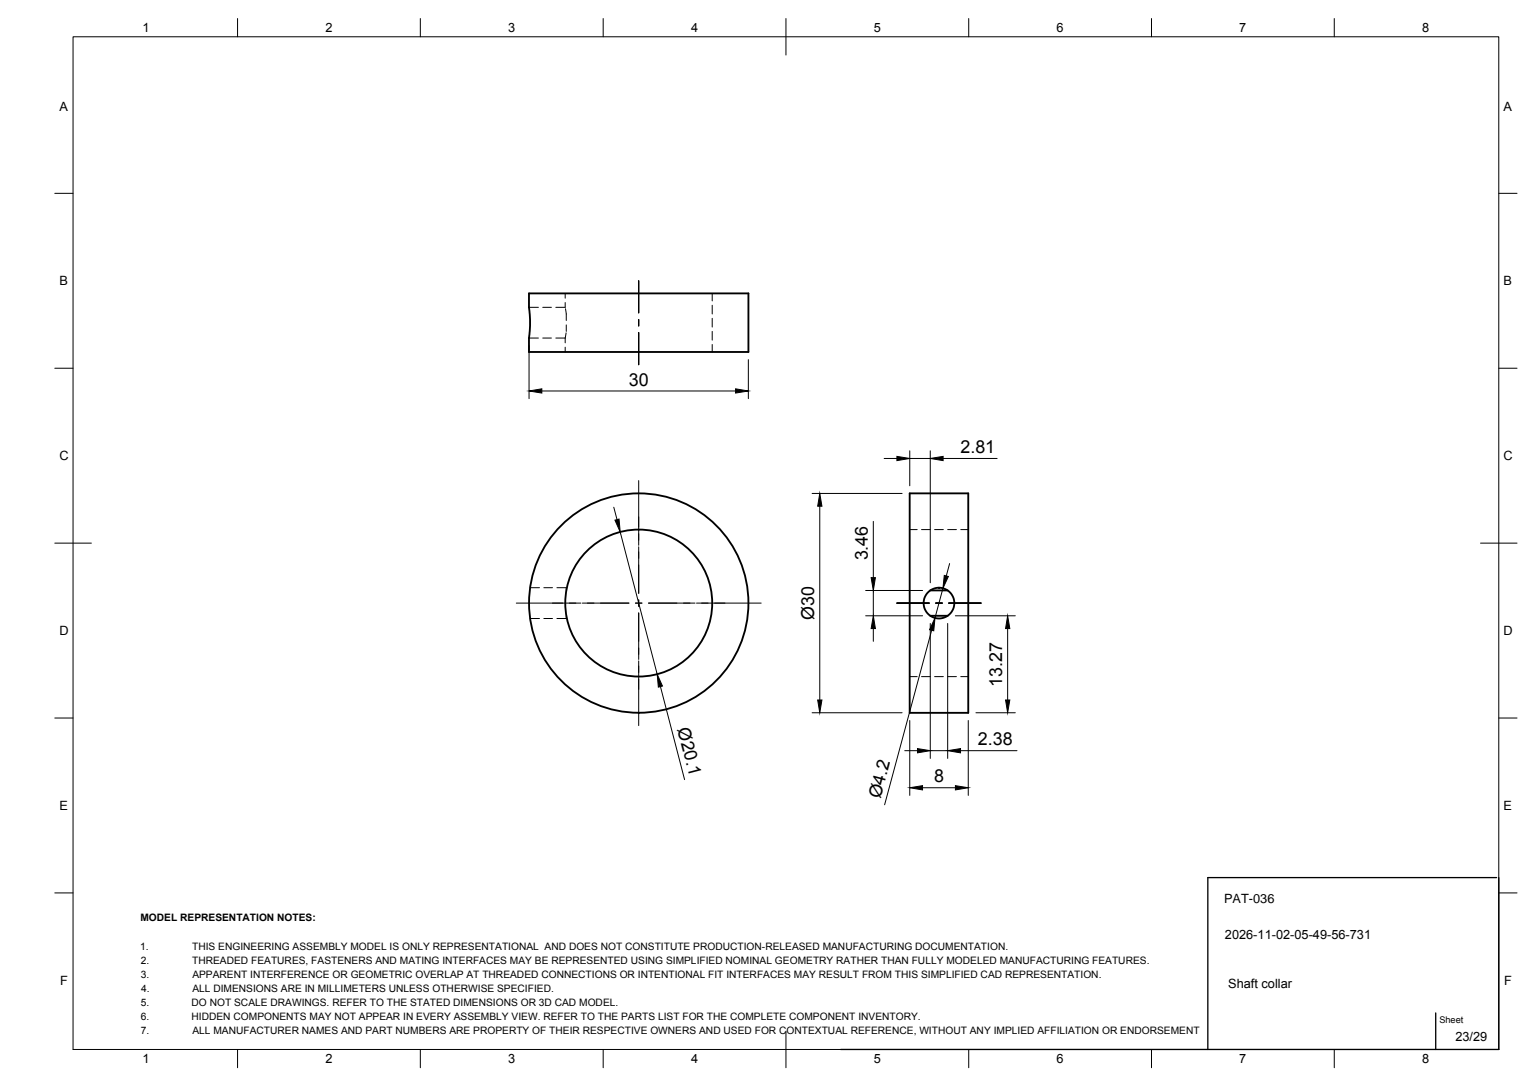
ISO-10303-21;
HEADER;
/* Generated by software containing ST-Developer
 * from STEP Tools, Inc. (www.steptools.com) 
 */

FILE_DESCRIPTION(
/* description */ ('Flange-mounted spindle'),
/* implementation_level */ '2;1');

FILE_NAME(
/* name */ 'Shaft collar.step',
/* time_stamp */ '2026-10-27T10:49:51-07:00',
/* author */ (''),
/* organization */ (''),
/* preprocessor_version */ 'ST-DEVELOPER v20.2',
/* originating_system */ 'Autodesk Translation Framework v15.17.0.0',
/* authorisation */ '');

FILE_SCHEMA (('AUTOMOTIVE_DESIGN { 1 0 10303 214 3 1 1 }'));
ENDSEC;

DATA;
#10=MECHANICAL_DESIGN_GEOMETRIC_PRESENTATION_REPRESENTATION('',(#355),#11764);
#235=B_SPLINE_CURVE_WITH_KNOTS('',3,(#10248,#10249,#10250,#10251,#10252,
#10253,#10254,#10255,#10256,#10257,#10258,#10259,#10260,#10261),
 .UNSPECIFIED.,.F.,.F.,(4,2,2,2,2,2,4),(0.75600573798701,0.793568827564647,
0.872922520054201,0.952276212543756,1.03162990503331,1.11098359752287,1.1485466871005),
 .UNSPECIFIED.);
#236=B_SPLINE_CURVE_WITH_KNOTS('',3,(#10267,#10268,#10269,#10270,#10271,
#10272,#10273,#10274,#10275,#10276,#10277,#10278,#10279,#10280,#10281,#10282,
#10283,#10284),.UNSPECIFIED.,.F.,.F.,(4,2,2,2,2,2,2,2,4),(0.,0.079216580773363,
0.158433161546726,0.23764869707457,0.316864232602414,0.396079768130259,
0.475295303658103,0.554511884431466,0.633728465204829),.UNSPECIFIED.);
#237=B_SPLINE_CURVE_WITH_KNOTS('',3,(#10285,#10286,#10287,#10288,#10289,
#10290,#10291,#10292,#10293,#10294,#10295,#10296,#10297,#10298,#10299,#10300,
#10301,#10302),.UNSPECIFIED.,.F.,.F.,(4,2,2,2,2,2,2,2,4),(0.633728465204829,
0.712945045978192,0.792161626751555,0.871377162279399,0.950592697807243,
1.02980823333509,1.10902376886293,1.18824034963629,1.26745693040966),
 .UNSPECIFIED.);
#238=B_SPLINE_CURVE_WITH_KNOTS('',3,(#10305,#10306,#10307,#10308,#10309,
#10310,#10311,#10312,#10313,#10314,#10315,#10316,#10317,#10318),
 .UNSPECIFIED.,.F.,.F.,(4,2,2,2,2,2,4),(0.121154929624507,0.158718019202143,
0.238071711691697,0.317425404181252,0.396779096670807,0.476132789160362,
0.513695878737997),.UNSPECIFIED.);
#300=SHAPE_REPRESENTATION_RELATIONSHIP('SRR','None',#11898,#327);
#327=ADVANCED_BREP_SHAPE_REPRESENTATION('',(#381),#11753);
#355=STYLED_ITEM('',(#12099),#381);
#381=MANIFOLD_SOLID_BREP('Body1',#6149);
#463=FACE_BOUND('',#1247,.T.);
#464=FACE_BOUND('',#1249,.T.);
#465=FACE_BOUND('',#1251,.T.);
#466=FACE_BOUND('',#1253,.T.);
#600=PLANE('',#6735);
#601=PLANE('',#6740);
#602=PLANE('',#6747);
#603=PLANE('',#6748);
#826=FACE_OUTER_BOUND('',#1243,.T.);
#827=FACE_OUTER_BOUND('',#1244,.T.);
#828=FACE_OUTER_BOUND('',#1245,.T.);
#829=FACE_OUTER_BOUND('',#1246,.T.);
#830=FACE_OUTER_BOUND('',#1248,.T.);
#831=FACE_OUTER_BOUND('',#1250,.T.);
#832=FACE_OUTER_BOUND('',#1252,.T.);
#1243=EDGE_LOOP('',(#4635,#4636));
#1244=EDGE_LOOP('',(#4637,#4638,#4639,#4640,#4641,#4642,#4643,#4644,#4645));
#1245=EDGE_LOOP('',(#4646,#4647,#4648));
#1246=EDGE_LOOP('',(#4649,#4650,#4651,#4652));
#1247=EDGE_LOOP('',(#4653,#4654,#4655,#4656));
#1248=EDGE_LOOP('',(#4657,#4658,#4659,#4660));
#1249=EDGE_LOOP('',(#4661,#4662));
#1250=EDGE_LOOP('',(#4663));
#1251=EDGE_LOOP('',(#4664));
#1252=EDGE_LOOP('',(#4665));
#1253=EDGE_LOOP('',(#4666));
#1669=LINE('',#10244,#2091);
#1670=LINE('',#10265,#2092);
#1671=LINE('',#10320,#2093);
#1672=LINE('',#10325,#2094);
#1673=LINE('',#10331,#2095);
#2091=VECTOR('',#7952,1.);
#2092=VECTOR('',#7959,0.21);
#2093=VECTOR('',#7964,1.);
#2094=VECTOR('',#7969,1.005);
#2095=VECTOR('',#7976,1.5);
#2424=CIRCLE('',#6736,0.21);
#2425=CIRCLE('',#6738,0.21);
#2426=CIRCLE('',#6739,0.21);
#2427=CIRCLE('',#6742,1.005);
#2428=CIRCLE('',#6743,1.005);
#2429=CIRCLE('',#6745,1.5);
#2430=CIRCLE('',#6746,1.5);
#2864=VERTEX_POINT('',#10242);
#2865=VERTEX_POINT('',#10243);
#2866=VERTEX_POINT('',#10247);
#2867=VERTEX_POINT('',#10262);
#2868=VERTEX_POINT('',#10264);
#2869=VERTEX_POINT('',#10266);
#2870=VERTEX_POINT('',#10303);
#2871=VERTEX_POINT('',#10322);
#2872=VERTEX_POINT('',#10324);
#2873=VERTEX_POINT('',#10328);
#2874=VERTEX_POINT('',#10330);
#3510=EDGE_CURVE('',#2864,#2865,#1669,.T.);
#3511=EDGE_CURVE('',#2864,#2865,#2424,.T.);
#3512=EDGE_CURVE('',#2866,#2864,#235,.T.);
#3513=EDGE_CURVE('',#2867,#2866,#2425,.T.);
#3514=EDGE_CURVE('',#2867,#2868,#1670,.T.);
#3515=EDGE_CURVE('',#2869,#2868,#236,.T.);
#3516=EDGE_CURVE('',#2868,#2869,#237,.T.);
#3517=EDGE_CURVE('',#2870,#2867,#2426,.T.);
#3518=EDGE_CURVE('',#2865,#2870,#238,.T.);
#3519=EDGE_CURVE('',#2870,#2866,#1671,.T.);
#3520=EDGE_CURVE('',#2871,#2871,#2427,.T.);
#3521=EDGE_CURVE('',#2871,#2872,#1672,.T.);
#3522=EDGE_CURVE('',#2872,#2872,#2428,.T.);
#3523=EDGE_CURVE('',#2873,#2873,#2429,.T.);
#3524=EDGE_CURVE('',#2873,#2874,#1673,.T.);
#3525=EDGE_CURVE('',#2874,#2874,#2430,.T.);
#4635=ORIENTED_EDGE('',*,*,#3510,.F.);
#4636=ORIENTED_EDGE('',*,*,#3511,.T.);
#4637=ORIENTED_EDGE('',*,*,#3512,.F.);
#4638=ORIENTED_EDGE('',*,*,#3513,.F.);
#4639=ORIENTED_EDGE('',*,*,#3514,.T.);
#4640=ORIENTED_EDGE('',*,*,#3515,.F.);
#4641=ORIENTED_EDGE('',*,*,#3516,.F.);
#4642=ORIENTED_EDGE('',*,*,#3514,.F.);
#4643=ORIENTED_EDGE('',*,*,#3517,.F.);
#4644=ORIENTED_EDGE('',*,*,#3518,.F.);
#4645=ORIENTED_EDGE('',*,*,#3511,.F.);
#4646=ORIENTED_EDGE('',*,*,#3519,.F.);
#4647=ORIENTED_EDGE('',*,*,#3517,.T.);
#4648=ORIENTED_EDGE('',*,*,#3513,.T.);
#4649=ORIENTED_EDGE('',*,*,#3520,.F.);
#4650=ORIENTED_EDGE('',*,*,#3521,.T.);
#4651=ORIENTED_EDGE('',*,*,#3522,.T.);
#4652=ORIENTED_EDGE('',*,*,#3521,.F.);
#4653=ORIENTED_EDGE('',*,*,#3518,.T.);
#4654=ORIENTED_EDGE('',*,*,#3519,.T.);
#4655=ORIENTED_EDGE('',*,*,#3512,.T.);
#4656=ORIENTED_EDGE('',*,*,#3510,.T.);
#4657=ORIENTED_EDGE('',*,*,#3523,.F.);
#4658=ORIENTED_EDGE('',*,*,#3524,.T.);
#4659=ORIENTED_EDGE('',*,*,#3525,.T.);
#4660=ORIENTED_EDGE('',*,*,#3524,.F.);
#4661=ORIENTED_EDGE('',*,*,#3515,.T.);
#4662=ORIENTED_EDGE('',*,*,#3516,.T.);
#4663=ORIENTED_EDGE('',*,*,#3523,.T.);
#4664=ORIENTED_EDGE('',*,*,#3520,.T.);
#4665=ORIENTED_EDGE('',*,*,#3525,.F.);
#4666=ORIENTED_EDGE('',*,*,#3522,.F.);
#5674=CYLINDRICAL_SURFACE('',#6737,0.21);
#5675=CYLINDRICAL_SURFACE('',#6741,1.005);
#5676=CYLINDRICAL_SURFACE('',#6744,1.5);
#5937=ADVANCED_FACE('',(#826),#600,.T.);
#5938=ADVANCED_FACE('',(#827),#5674,.F.);
#5939=ADVANCED_FACE('',(#828),#601,.T.);
#5940=ADVANCED_FACE('',(#829,#463),#5675,.F.);
#5941=ADVANCED_FACE('',(#830,#464),#5676,.T.);
#5942=ADVANCED_FACE('',(#831,#465),#602,.T.);
#5943=ADVANCED_FACE('',(#832,#466),#603,.F.);
#6149=CLOSED_SHELL('',(#5937,#5938,#5939,#5940,#5941,#5942,#5943));
#6734=AXIS2_PLACEMENT_3D('',#10240,#7948,#7949);
#6735=AXIS2_PLACEMENT_3D('',#10241,#7950,#7951);
#6736=AXIS2_PLACEMENT_3D('',#10245,#7953,#7954);
#6737=AXIS2_PLACEMENT_3D('',#10246,#7955,#7956);
#6738=AXIS2_PLACEMENT_3D('',#10263,#7957,#7958);
#6739=AXIS2_PLACEMENT_3D('',#10304,#7960,#7961);
#6740=AXIS2_PLACEMENT_3D('',#10319,#7962,#7963);
#6741=AXIS2_PLACEMENT_3D('',#10321,#7965,#7966);
#6742=AXIS2_PLACEMENT_3D('',#10323,#7967,#7968);
#6743=AXIS2_PLACEMENT_3D('',#10326,#7970,#7971);
#6744=AXIS2_PLACEMENT_3D('',#10327,#7972,#7973);
#6745=AXIS2_PLACEMENT_3D('',#10329,#7974,#7975);
#6746=AXIS2_PLACEMENT_3D('',#10332,#7977,#7978);
#6747=AXIS2_PLACEMENT_3D('',#10333,#7979,#7980);
#6748=AXIS2_PLACEMENT_3D('',#10334,#7981,#7982);
#7948=DIRECTION('axis',(0.,0.,1.));
#7949=DIRECTION('refdir',(1.,0.,0.));
#7950=DIRECTION('center_axis',(0.,0.,1.));
#7951=DIRECTION('ref_axis',(1.,0.,0.));
#7952=DIRECTION('',(0.,1.,0.));
#7953=DIRECTION('center_axis',(0.,0.,1.));
#7954=DIRECTION('ref_axis',(1.,0.,0.));
#7955=DIRECTION('center_axis',(0.,0.,1.));
#7956=DIRECTION('ref_axis',(1.,0.,0.));
#7957=DIRECTION('center_axis',(0.,0.,1.));
#7958=DIRECTION('ref_axis',(1.,0.,0.));
#7959=DIRECTION('',(0.,0.,1.));
#7960=DIRECTION('center_axis',(0.,0.,1.));
#7961=DIRECTION('ref_axis',(1.,0.,0.));
#7962=DIRECTION('center_axis',(0.,0.,1.));
#7963=DIRECTION('ref_axis',(1.,0.,0.));
#7964=DIRECTION('',(0.,-1.,0.));
#7965=DIRECTION('center_axis',(0.,1.,0.));
#7966=DIRECTION('ref_axis',(1.,0.,0.));
#7967=DIRECTION('center_axis',(0.,-1.,0.));
#7968=DIRECTION('ref_axis',(1.,0.,0.));
#7969=DIRECTION('',(0.,-1.,0.));
#7970=DIRECTION('center_axis',(0.,-1.,0.));
#7971=DIRECTION('ref_axis',(1.,0.,0.));
#7972=DIRECTION('center_axis',(0.,1.,0.));
#7973=DIRECTION('ref_axis',(1.,0.,0.));
#7974=DIRECTION('center_axis',(0.,1.,0.));
#7975=DIRECTION('ref_axis',(1.,0.,0.));
#7976=DIRECTION('',(0.,-1.,0.));
#7977=DIRECTION('center_axis',(0.,1.,0.));
#7978=DIRECTION('ref_axis',(1.,0.,0.));
#7979=DIRECTION('center_axis',(0.,1.,0.));
#7980=DIRECTION('ref_axis',(1.,0.,0.));
#7981=DIRECTION('center_axis',(0.,1.,0.));
#7982=DIRECTION('ref_axis',(1.,0.,0.));
#10240=CARTESIAN_POINT('',(0.,0.,0.));
#10241=CARTESIAN_POINT('Origin',(0.,-1.25,8.99));
#10242=CARTESIAN_POINT('',(0.172988438920061,-1.36905880899791,8.99));
#10243=CARTESIAN_POINT('',(0.172988438920061,-1.13094119100209,8.99));
#10244=CARTESIAN_POINT('',(0.172988438920061,-1.65,8.99));
#10245=CARTESIAN_POINT('Origin',(0.,-1.25,8.99));
#10246=CARTESIAN_POINT('Origin',(0.,-1.25,8.99));
#10247=CARTESIAN_POINT('',(-0.172988438920061,-1.36905880899791,8.99));
#10248=CARTESIAN_POINT('Ctrl Pts',(-0.172988438920061,-1.36905880899791,
8.99));
#10249=CARTESIAN_POINT('Ctrl Pts',(-0.165594865311318,-1.37980142239529,
8.99129192197638));
#10250=CARTESIAN_POINT('Ctrl Pts',(-0.157297138725608,-1.38968770937274,
8.99265394943905));
#10251=CARTESIAN_POINT('Ctrl Pts',(-0.129892073845076,-1.41709277425327,
8.9967480843909));
#10252=CARTESIAN_POINT('Ctrl Pts',(-0.106330167759284,-1.43324205633295,
8.99969589327638));
#10253=CARTESIAN_POINT('Ctrl Pts',(-0.0546129046324105,-1.45469779396491,
9.00385029472357));
#10254=CARTESIAN_POINT('Ctrl Pts',(-0.0264512308298517,-1.46,9.005));
#10255=CARTESIAN_POINT('Ctrl Pts',(0.0264512308298516,-1.46,9.005));
#10256=CARTESIAN_POINT('Ctrl Pts',(0.0546129046324105,-1.45469779396491,
9.00385029472357));
#10257=CARTESIAN_POINT('Ctrl Pts',(0.106330167759284,-1.43324205633295,
8.99969589327638));
#10258=CARTESIAN_POINT('Ctrl Pts',(0.129892073845076,-1.41709277425327,
8.9967480843909));
#10259=CARTESIAN_POINT('Ctrl Pts',(0.157297138725608,-1.38968770937274,
8.99265394943905));
#10260=CARTESIAN_POINT('Ctrl Pts',(0.165594865311318,-1.37980142239529,
8.99129192197638));
#10261=CARTESIAN_POINT('Ctrl Pts',(0.172988438920061,-1.36905880899791,
8.99));
#10262=CARTESIAN_POINT('',(-0.21,-1.25,8.99));
#10263=CARTESIAN_POINT('Origin',(0.,-1.25,8.99));
#10264=CARTESIAN_POINT('',(-0.21,-1.25,9.48522725533839));
#10265=CARTESIAN_POINT('',(-0.21,-1.25,8.99));
#10266=CARTESIAN_POINT('',(0.21,-1.25,9.48522725533839));
#10267=CARTESIAN_POINT('Ctrl Pts',(0.21,-1.25,9.48522725533839));
#10268=CARTESIAN_POINT('Ctrl Pts',(0.21,-1.27640552692445,9.48522725533839));
#10269=CARTESIAN_POINT('Ctrl Pts',(0.204715737269596,-1.30454707409071,
9.48600415954412));
#10270=CARTESIAN_POINT('Ctrl Pts',(0.183273763036331,-1.35627626890513,
9.48880073282317));
#10271=CARTESIAN_POINT('Ctrl Pts',(0.167117923970394,-1.37986692412796,
9.49077897157582));
#10272=CARTESIAN_POINT('Ctrl Pts',(0.129867169887369,-1.41711767821098,
9.49448481141327));
#10273=CARTESIAN_POINT('Ctrl Pts',(0.106276408305765,-1.43327371000135,
9.49645455657129));
#10274=CARTESIAN_POINT('Ctrl Pts',(0.0545468514059002,-1.45471582482622,
9.49923165515646));
#10275=CARTESIAN_POINT('Ctrl Pts',(0.0264051785092814,-1.46,9.5));
#10276=CARTESIAN_POINT('Ctrl Pts',(-0.0264051785092814,-1.46,9.5));
#10277=CARTESIAN_POINT('Ctrl Pts',(-0.0545468514059001,-1.45471582482622,
9.49923165515646));
#10278=CARTESIAN_POINT('Ctrl Pts',(-0.106276408305765,-1.43327371000135,
9.49645455657129));
#10279=CARTESIAN_POINT('Ctrl Pts',(-0.129867169887369,-1.41711767821098,
9.49448481141327));
#10280=CARTESIAN_POINT('Ctrl Pts',(-0.167117923970394,-1.37986692412796,
9.49077897157582));
#10281=CARTESIAN_POINT('Ctrl Pts',(-0.183273763036331,-1.35627626890513,
9.48880073282317));
#10282=CARTESIAN_POINT('Ctrl Pts',(-0.204715737269596,-1.30454707409071,
9.48600415954412));
#10283=CARTESIAN_POINT('Ctrl Pts',(-0.21,-1.27640552692445,9.48522725533839));
#10284=CARTESIAN_POINT('Ctrl Pts',(-0.21,-1.25,9.48522725533839));
#10285=CARTESIAN_POINT('Ctrl Pts',(-0.21,-1.25,9.48522725533839));
#10286=CARTESIAN_POINT('Ctrl Pts',(-0.21,-1.22359447307555,9.48522725533839));
#10287=CARTESIAN_POINT('Ctrl Pts',(-0.204715737269596,-1.19545292590929,
9.48600415954412));
#10288=CARTESIAN_POINT('Ctrl Pts',(-0.183273763036331,-1.14372373109487,
9.48880073282317));
#10289=CARTESIAN_POINT('Ctrl Pts',(-0.167117923970394,-1.12013307587204,
9.49077897157582));
#10290=CARTESIAN_POINT('Ctrl Pts',(-0.129867169887369,-1.08288232178902,
9.49448481141327));
#10291=CARTESIAN_POINT('Ctrl Pts',(-0.106276408305765,-1.06672628999865,
9.49645455657129));
#10292=CARTESIAN_POINT('Ctrl Pts',(-0.0545468514059002,-1.04528417517378,
9.49923165515646));
#10293=CARTESIAN_POINT('Ctrl Pts',(-0.0264051785092814,-1.04,9.5));
#10294=CARTESIAN_POINT('Ctrl Pts',(0.0264051785092814,-1.04,9.5));
#10295=CARTESIAN_POINT('Ctrl Pts',(0.0545468514059002,-1.04528417517378,
9.49923165515645));
#10296=CARTESIAN_POINT('Ctrl Pts',(0.106276408305765,-1.06672628999865,
9.49645455657129));
#10297=CARTESIAN_POINT('Ctrl Pts',(0.129867169887369,-1.08288232178902,
9.49448481141327));
#10298=CARTESIAN_POINT('Ctrl Pts',(0.167117923970394,-1.12013307587204,
9.49077897157582));
#10299=CARTESIAN_POINT('Ctrl Pts',(0.183273763036332,-1.14372373109487,
9.48880073282317));
#10300=CARTESIAN_POINT('Ctrl Pts',(0.204715737269596,-1.19545292590929,
9.48600415954412));
#10301=CARTESIAN_POINT('Ctrl Pts',(0.21,-1.22359447307555,9.48522725533839));
#10302=CARTESIAN_POINT('Ctrl Pts',(0.21,-1.25,9.48522725533839));
#10303=CARTESIAN_POINT('',(-0.172988438920061,-1.13094119100209,8.99));
#10304=CARTESIAN_POINT('Origin',(0.,-1.25,8.99));
#10305=CARTESIAN_POINT('Ctrl Pts',(0.172988438920061,-1.13094119100209,
8.99));
#10306=CARTESIAN_POINT('Ctrl Pts',(0.165594865311318,-1.12019857760471,
8.99129192197638));
#10307=CARTESIAN_POINT('Ctrl Pts',(0.157297138725608,-1.11031229062726,
8.99265394943905));
#10308=CARTESIAN_POINT('Ctrl Pts',(0.129892073845076,-1.08290722574673,
8.9967480843909));
#10309=CARTESIAN_POINT('Ctrl Pts',(0.106330167759284,-1.06675794366705,
8.99969589327638));
#10310=CARTESIAN_POINT('Ctrl Pts',(0.0546129046324105,-1.04530220603509,
9.00385029472357));
#10311=CARTESIAN_POINT('Ctrl Pts',(0.0264512308298516,-1.04,9.005));
#10312=CARTESIAN_POINT('Ctrl Pts',(-0.0264512308298516,-1.04,9.005));
#10313=CARTESIAN_POINT('Ctrl Pts',(-0.0546129046324105,-1.04530220603509,
9.00385029472357));
#10314=CARTESIAN_POINT('Ctrl Pts',(-0.106330167759284,-1.06675794366705,
8.99969589327638));
#10315=CARTESIAN_POINT('Ctrl Pts',(-0.129892073845076,-1.08290722574673,
8.9967480843909));
#10316=CARTESIAN_POINT('Ctrl Pts',(-0.157297138725608,-1.11031229062726,
8.99265394943905));
#10317=CARTESIAN_POINT('Ctrl Pts',(-0.165594865311318,-1.12019857760471,
8.99129192197638));
#10318=CARTESIAN_POINT('Ctrl Pts',(-0.172988438920061,-1.13094119100209,
8.99));
#10319=CARTESIAN_POINT('Origin',(0.,-1.25,8.99));
#10320=CARTESIAN_POINT('',(-0.172988438920061,-1.65,8.99));
#10321=CARTESIAN_POINT('Origin',(0.,-1.65,8.));
#10322=CARTESIAN_POINT('',(-1.005,-0.85,8.));
#10323=CARTESIAN_POINT('Origin',(0.,-0.85,8.));
#10324=CARTESIAN_POINT('',(-1.005,-1.65,8.));
#10325=CARTESIAN_POINT('',(-1.005,-1.65,8.));
#10326=CARTESIAN_POINT('Origin',(0.,-1.65,8.));
#10327=CARTESIAN_POINT('Origin',(0.,-1.65,8.));
#10328=CARTESIAN_POINT('',(-1.5,-0.85,8.));
#10329=CARTESIAN_POINT('Origin',(0.,-0.85,8.));
#10330=CARTESIAN_POINT('',(-1.5,-1.65,8.));
#10331=CARTESIAN_POINT('',(-1.5,-1.65,8.));
#10332=CARTESIAN_POINT('Origin',(0.,-1.65,8.));
#10333=CARTESIAN_POINT('Origin',(0.,-0.85,8.));
#10334=CARTESIAN_POINT('Origin',(0.,-1.65,8.));
#11721=UNCERTAINTY_MEASURE_WITH_UNIT(LENGTH_MEASURE(0.001),#11765,
'DISTANCE_ACCURACY_VALUE',
'Maximum model space distance between geometric entities at asserted c
onnectivities');
#11732=UNCERTAINTY_MEASURE_WITH_UNIT(LENGTH_MEASURE(0.001),#11765,
'DISTANCE_ACCURACY_VALUE',
'Maximum model space distance between geometric entities at asserted c
onnectivities');
#11753=(
GEOMETRIC_REPRESENTATION_CONTEXT(3)
GLOBAL_UNCERTAINTY_ASSIGNED_CONTEXT((#11721))
GLOBAL_UNIT_ASSIGNED_CONTEXT((#11765,#11767,#11768))
REPRESENTATION_CONTEXT('','3D')
);
#11764=(
GEOMETRIC_REPRESENTATION_CONTEXT(3)
GLOBAL_UNCERTAINTY_ASSIGNED_CONTEXT((#11732))
GLOBAL_UNIT_ASSIGNED_CONTEXT((#11765,#11767,#11768))
REPRESENTATION_CONTEXT('','3D')
);
#11765=(
LENGTH_UNIT()
NAMED_UNIT(*)
SI_UNIT(.CENTI.,.METRE.)
);
#11767=(
NAMED_UNIT(*)
PLANE_ANGLE_UNIT()
SI_UNIT($,.RADIAN.)
);
#11768=(
NAMED_UNIT(*)
SI_UNIT($,.STERADIAN.)
SOLID_ANGLE_UNIT()
);
#11789=SHAPE_DEFINITION_REPRESENTATION(#11822,#11898);
#11822=PRODUCT_DEFINITION_SHAPE('',$,#11930);
#11898=SHAPE_REPRESENTATION('',(#6734),#11753);
#11909=PRODUCT_DEFINITION_CONTEXT('part definition',#12004,'design');
#11930=PRODUCT_DEFINITION('Shaft collar','Shaft collar',#11961,#11909);
#11961=PRODUCT_DEFINITION_FORMATION('',$,#12026);
#12004=APPLICATION_CONTEXT(
'Core Data for Automotive Mechanical Design Process');
#12005=PRODUCT_CONTEXT('part definition',#12004,'mechanical');
#12026=PRODUCT('Shaft collar','Shaft collar','Shaft collar',(#12005));
#12093=COLOUR_RGB('Grey',0.48,0.52,0.57);
#12094=FILL_AREA_STYLE_COLOUR('',#12093);
#12095=FILL_AREA_STYLE('',(#12094));
#12096=SURFACE_STYLE_FILL_AREA(#12095);
#12097=SURFACE_SIDE_STYLE('',(#12096));
#12098=SURFACE_STYLE_USAGE(.BOTH.,#12097);
#12099=PRESENTATION_STYLE_ASSIGNMENT((#12098));
ENDSEC;
END-ISO-10303-21;
